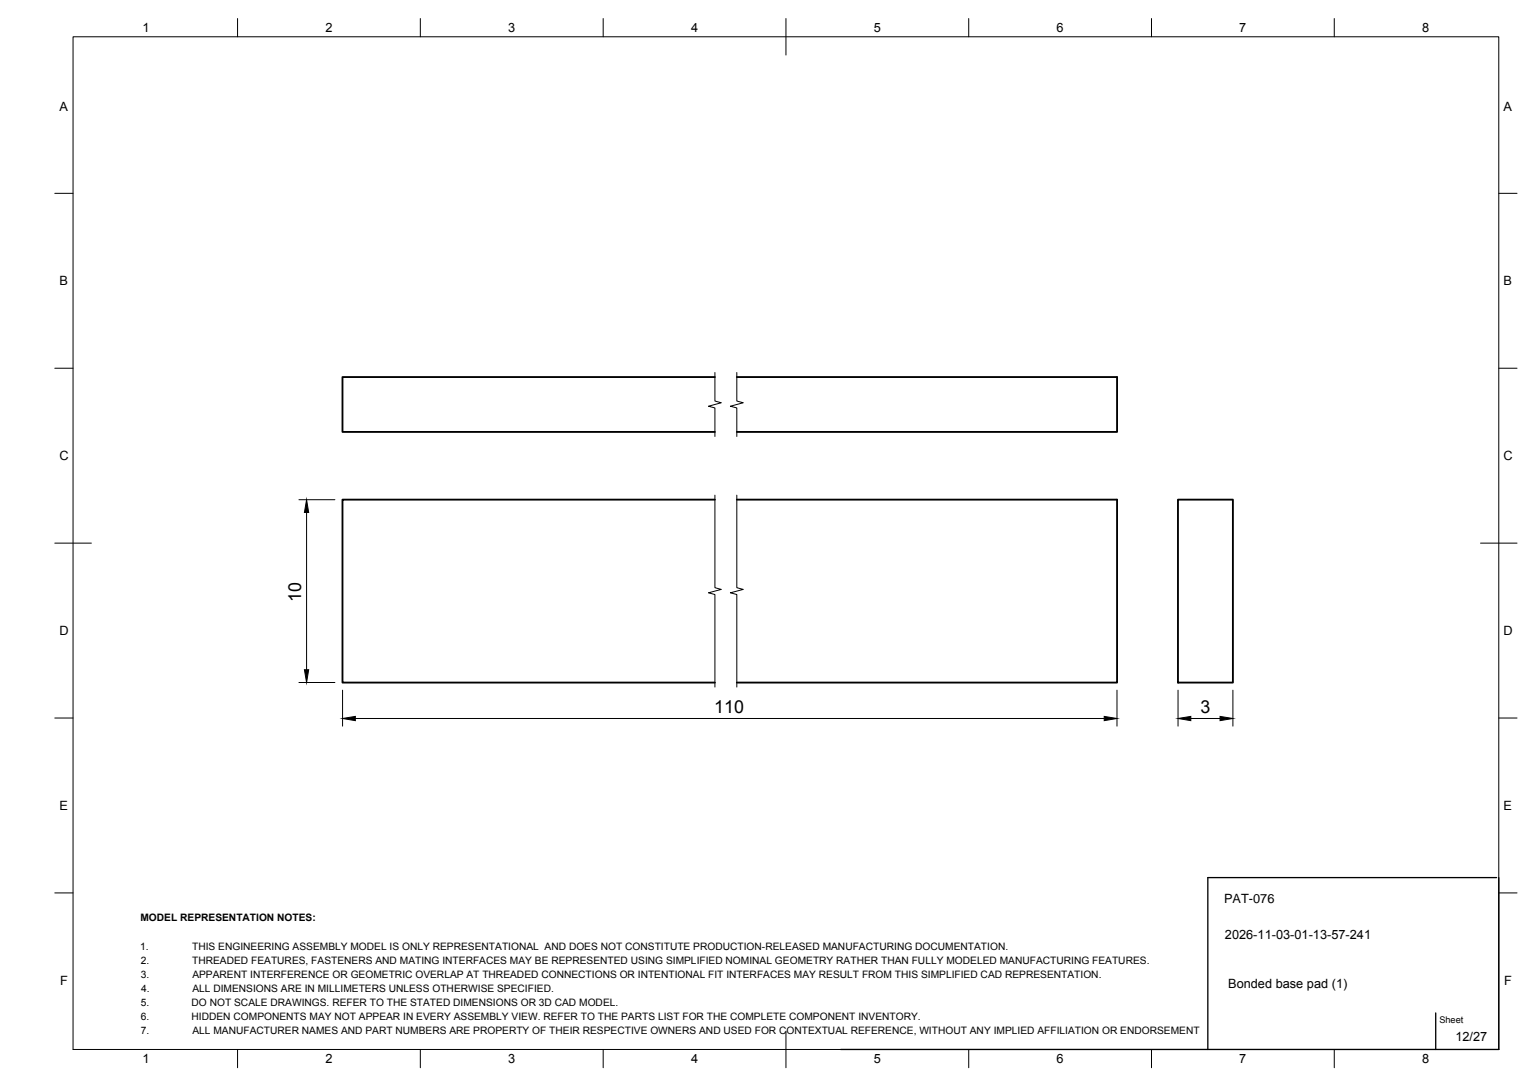
ISO-10303-21;
HEADER;
/* Generated by software containing ST-Developer
 * from STEP Tools, Inc. (www.steptools.com) 
 */

FILE_DESCRIPTION(
/* description */ ('Overhung pulley bearing cartridge'),
/* implementation_level */ '2;1');

FILE_NAME(
/* name */ 'Bonded base pad (1).step',
/* time_stamp */ '2026-10-28T03:22:33-07:00',
/* author */ (''),
/* organization */ (''),
/* preprocessor_version */ 'ST-DEVELOPER v20.2',
/* originating_system */ 'Autodesk Translation Framework v15.17.0.0',
/* authorisation */ '');

FILE_SCHEMA (('AUTOMOTIVE_DESIGN { 1 0 10303 214 3 1 1 }'));
ENDSEC;

DATA;
#10=MECHANICAL_DESIGN_GEOMETRIC_PRESENTATION_REPRESENTATION('',(#290),#10963);
#246=SHAPE_REPRESENTATION_RELATIONSHIP('SRR','None',#11066,#268);
#268=ADVANCED_BREP_SHAPE_REPRESENTATION('',(#320),#10946);
#290=STYLED_ITEM('',(#11232),#320);
#320=MANIFOLD_SOLID_BREP('Body1',#5657);
#485=PLANE('',#6105);
#486=PLANE('',#6106);
#487=PLANE('',#6107);
#488=PLANE('',#6108);
#489=PLANE('',#6109);
#490=PLANE('',#6110);
#665=FACE_OUTER_BOUND('',#1049,.T.);
#666=FACE_OUTER_BOUND('',#1050,.T.);
#667=FACE_OUTER_BOUND('',#1051,.T.);
#668=FACE_OUTER_BOUND('',#1052,.T.);
#669=FACE_OUTER_BOUND('',#1053,.T.);
#670=FACE_OUTER_BOUND('',#1054,.T.);
#1049=EDGE_LOOP('',(#4011,#4012,#4013,#4014));
#1050=EDGE_LOOP('',(#4015,#4016,#4017,#4018));
#1051=EDGE_LOOP('',(#4019,#4020,#4021,#4022));
#1052=EDGE_LOOP('',(#4023,#4024,#4025,#4026));
#1053=EDGE_LOOP('',(#4027,#4028,#4029,#4030));
#1054=EDGE_LOOP('',(#4031,#4032,#4033,#4034));
#1425=LINE('',#8954,#1767);
#1426=LINE('',#8956,#1768);
#1427=LINE('',#8958,#1769);
#1428=LINE('',#8959,#1770);
#1429=LINE('',#8962,#1771);
#1430=LINE('',#8964,#1772);
#1431=LINE('',#8965,#1773);
#1432=LINE('',#8968,#1774);
#1433=LINE('',#8970,#1775);
#1434=LINE('',#8971,#1776);
#1435=LINE('',#8973,#1777);
#1436=LINE('',#8974,#1778);
#1767=VECTOR('',#7147,1.);
#1768=VECTOR('',#7148,1.);
#1769=VECTOR('',#7149,1.);
#1770=VECTOR('',#7150,1.);
#1771=VECTOR('',#7153,1.);
#1772=VECTOR('',#7154,1.);
#1773=VECTOR('',#7155,1.);
#1774=VECTOR('',#7158,1.);
#1775=VECTOR('',#7159,1.);
#1776=VECTOR('',#7160,1.);
#1777=VECTOR('',#7163,1.);
#1778=VECTOR('',#7164,1.);
#2501=VERTEX_POINT('',#8952);
#2502=VERTEX_POINT('',#8953);
#2503=VERTEX_POINT('',#8955);
#2504=VERTEX_POINT('',#8957);
#2505=VERTEX_POINT('',#8961);
#2506=VERTEX_POINT('',#8963);
#2507=VERTEX_POINT('',#8967);
#2508=VERTEX_POINT('',#8969);
#3075=EDGE_CURVE('',#2501,#2502,#1425,.T.);
#3076=EDGE_CURVE('',#2502,#2503,#1426,.T.);
#3077=EDGE_CURVE('',#2504,#2503,#1427,.T.);
#3078=EDGE_CURVE('',#2501,#2504,#1428,.T.);
#3079=EDGE_CURVE('',#2505,#2501,#1429,.T.);
#3080=EDGE_CURVE('',#2506,#2504,#1430,.T.);
#3081=EDGE_CURVE('',#2505,#2506,#1431,.T.);
#3082=EDGE_CURVE('',#2507,#2505,#1432,.T.);
#3083=EDGE_CURVE('',#2508,#2506,#1433,.T.);
#3084=EDGE_CURVE('',#2507,#2508,#1434,.T.);
#3085=EDGE_CURVE('',#2502,#2507,#1435,.T.);
#3086=EDGE_CURVE('',#2503,#2508,#1436,.T.);
#4011=ORIENTED_EDGE('',*,*,#3075,.T.);
#4012=ORIENTED_EDGE('',*,*,#3076,.T.);
#4013=ORIENTED_EDGE('',*,*,#3077,.F.);
#4014=ORIENTED_EDGE('',*,*,#3078,.F.);
#4015=ORIENTED_EDGE('',*,*,#3079,.T.);
#4016=ORIENTED_EDGE('',*,*,#3078,.T.);
#4017=ORIENTED_EDGE('',*,*,#3080,.F.);
#4018=ORIENTED_EDGE('',*,*,#3081,.F.);
#4019=ORIENTED_EDGE('',*,*,#3082,.T.);
#4020=ORIENTED_EDGE('',*,*,#3081,.T.);
#4021=ORIENTED_EDGE('',*,*,#3083,.F.);
#4022=ORIENTED_EDGE('',*,*,#3084,.F.);
#4023=ORIENTED_EDGE('',*,*,#3085,.T.);
#4024=ORIENTED_EDGE('',*,*,#3084,.T.);
#4025=ORIENTED_EDGE('',*,*,#3086,.F.);
#4026=ORIENTED_EDGE('',*,*,#3076,.F.);
#4027=ORIENTED_EDGE('',*,*,#3086,.T.);
#4028=ORIENTED_EDGE('',*,*,#3083,.T.);
#4029=ORIENTED_EDGE('',*,*,#3080,.T.);
#4030=ORIENTED_EDGE('',*,*,#3077,.T.);
#4031=ORIENTED_EDGE('',*,*,#3085,.F.);
#4032=ORIENTED_EDGE('',*,*,#3075,.F.);
#4033=ORIENTED_EDGE('',*,*,#3079,.F.);
#4034=ORIENTED_EDGE('',*,*,#3082,.F.);
#5409=ADVANCED_FACE('',(#665),#485,.T.);
#5410=ADVANCED_FACE('',(#666),#486,.T.);
#5411=ADVANCED_FACE('',(#667),#487,.T.);
#5412=ADVANCED_FACE('',(#668),#488,.T.);
#5413=ADVANCED_FACE('',(#669),#489,.T.);
#5414=ADVANCED_FACE('',(#670),#490,.F.);
#5657=CLOSED_SHELL('',(#5409,#5410,#5411,#5412,#5413,#5414));
#6104=AXIS2_PLACEMENT_3D('',#8950,#7143,#7144);
#6105=AXIS2_PLACEMENT_3D('',#8951,#7145,#7146);
#6106=AXIS2_PLACEMENT_3D('',#8960,#7151,#7152);
#6107=AXIS2_PLACEMENT_3D('',#8966,#7156,#7157);
#6108=AXIS2_PLACEMENT_3D('',#8972,#7161,#7162);
#6109=AXIS2_PLACEMENT_3D('',#8975,#7165,#7166);
#6110=AXIS2_PLACEMENT_3D('',#8976,#7167,#7168);
#7143=DIRECTION('axis',(0.,0.,1.));
#7144=DIRECTION('refdir',(1.,0.,0.));
#7145=DIRECTION('center_axis',(0.,1.,0.));
#7146=DIRECTION('ref_axis',(-1.,0.,0.));
#7147=DIRECTION('',(-1.,0.,0.));
#7148=DIRECTION('',(0.,0.,1.));
#7149=DIRECTION('',(-1.,0.,0.));
#7150=DIRECTION('',(0.,0.,1.));
#7151=DIRECTION('center_axis',(1.,0.,0.));
#7152=DIRECTION('ref_axis',(0.,1.,0.));
#7153=DIRECTION('',(0.,1.,0.));
#7154=DIRECTION('',(0.,1.,0.));
#7155=DIRECTION('',(0.,0.,1.));
#7156=DIRECTION('center_axis',(0.,-1.,0.));
#7157=DIRECTION('ref_axis',(1.,0.,0.));
#7158=DIRECTION('',(1.,0.,0.));
#7159=DIRECTION('',(1.,0.,0.));
#7160=DIRECTION('',(0.,0.,1.));
#7161=DIRECTION('center_axis',(-1.,0.,0.));
#7162=DIRECTION('ref_axis',(0.,-1.,0.));
#7163=DIRECTION('',(0.,-1.,0.));
#7164=DIRECTION('',(0.,-1.,0.));
#7165=DIRECTION('center_axis',(0.,0.,1.));
#7166=DIRECTION('ref_axis',(1.,0.,0.));
#7167=DIRECTION('center_axis',(0.,0.,1.));
#7168=DIRECTION('ref_axis',(1.,0.,0.));
#8950=CARTESIAN_POINT('',(0.,0.,0.));
#8951=CARTESIAN_POINT('Origin',(5.5,7.,-0.3));
#8952=CARTESIAN_POINT('',(5.5,7.,-0.3));
#8953=CARTESIAN_POINT('',(-5.5,7.,-0.3));
#8954=CARTESIAN_POINT('',(5.5,7.,-0.3));
#8955=CARTESIAN_POINT('',(-5.5,7.,0.));
#8956=CARTESIAN_POINT('',(-5.5,7.,-0.3));
#8957=CARTESIAN_POINT('',(5.5,7.,0.));
#8958=CARTESIAN_POINT('',(5.5,7.,0.));
#8959=CARTESIAN_POINT('',(5.5,7.,-0.3));
#8960=CARTESIAN_POINT('Origin',(5.5,6.,-0.3));
#8961=CARTESIAN_POINT('',(5.5,6.,-0.3));
#8962=CARTESIAN_POINT('',(5.5,6.,-0.3));
#8963=CARTESIAN_POINT('',(5.5,6.,0.));
#8964=CARTESIAN_POINT('',(5.5,6.,0.));
#8965=CARTESIAN_POINT('',(5.5,6.,-0.3));
#8966=CARTESIAN_POINT('Origin',(-5.5,6.,-0.3));
#8967=CARTESIAN_POINT('',(-5.5,6.,-0.3));
#8968=CARTESIAN_POINT('',(-5.5,6.,-0.3));
#8969=CARTESIAN_POINT('',(-5.5,6.,0.));
#8970=CARTESIAN_POINT('',(-5.5,6.,0.));
#8971=CARTESIAN_POINT('',(-5.5,6.,-0.3));
#8972=CARTESIAN_POINT('Origin',(-5.5,7.,-0.3));
#8973=CARTESIAN_POINT('',(-5.5,7.,-0.3));
#8974=CARTESIAN_POINT('',(-5.5,7.,0.));
#8975=CARTESIAN_POINT('Origin',(0.,6.5,0.));
#8976=CARTESIAN_POINT('Origin',(0.,6.5,-0.3));
#10919=UNCERTAINTY_MEASURE_WITH_UNIT(LENGTH_MEASURE(0.001),#10964,
'DISTANCE_ACCURACY_VALUE',
'Maximum model space distance between geometric entities at asserted c
onnectivities');
#10936=UNCERTAINTY_MEASURE_WITH_UNIT(LENGTH_MEASURE(0.001),#10964,
'DISTANCE_ACCURACY_VALUE',
'Maximum model space distance between geometric entities at asserted c
onnectivities');
#10946=(
GEOMETRIC_REPRESENTATION_CONTEXT(3)
GLOBAL_UNCERTAINTY_ASSIGNED_CONTEXT((#10919))
GLOBAL_UNIT_ASSIGNED_CONTEXT((#10964,#10966,#10967))
REPRESENTATION_CONTEXT('','3D')
);
#10963=(
GEOMETRIC_REPRESENTATION_CONTEXT(3)
GLOBAL_UNCERTAINTY_ASSIGNED_CONTEXT((#10936))
GLOBAL_UNIT_ASSIGNED_CONTEXT((#10964,#10966,#10967))
REPRESENTATION_CONTEXT('','3D')
);
#10964=(
LENGTH_UNIT()
NAMED_UNIT(*)
SI_UNIT(.CENTI.,.METRE.)
);
#10966=(
NAMED_UNIT(*)
PLANE_ANGLE_UNIT()
SI_UNIT($,.RADIAN.)
);
#10967=(
NAMED_UNIT(*)
SI_UNIT($,.STERADIAN.)
SOLID_ANGLE_UNIT()
);
#10977=SHAPE_DEFINITION_REPRESENTATION(#11003,#11066);
#11003=PRODUCT_DEFINITION_SHAPE('',$,#11093);
#11066=SHAPE_REPRESENTATION('',(#6104),#10946);
#11083=PRODUCT_DEFINITION_CONTEXT('part definition',#11163,'design');
#11093=PRODUCT_DEFINITION('Bonded base pad (1)','Bonded base pad (1)',#11119,
#11083);
#11119=PRODUCT_DEFINITION_FORMATION('',$,#11174);
#11163=APPLICATION_CONTEXT(
'Core Data for Automotive Mechanical Design Process');
#11164=PRODUCT_CONTEXT('part definition',#11163,'mechanical');
#11174=PRODUCT('Bonded base pad (1)','Bonded base pad (1)',
'Bonded base pad (1)',(#11164));
#11226=COLOUR_RGB('Dark Blue',0.08,0.2,0.34);
#11227=FILL_AREA_STYLE_COLOUR('',#11226);
#11228=FILL_AREA_STYLE('',(#11227));
#11229=SURFACE_STYLE_FILL_AREA(#11228);
#11230=SURFACE_SIDE_STYLE('',(#11229));
#11231=SURFACE_STYLE_USAGE(.BOTH.,#11230);
#11232=PRESENTATION_STYLE_ASSIGNMENT((#11231));
ENDSEC;
END-ISO-10303-21;
